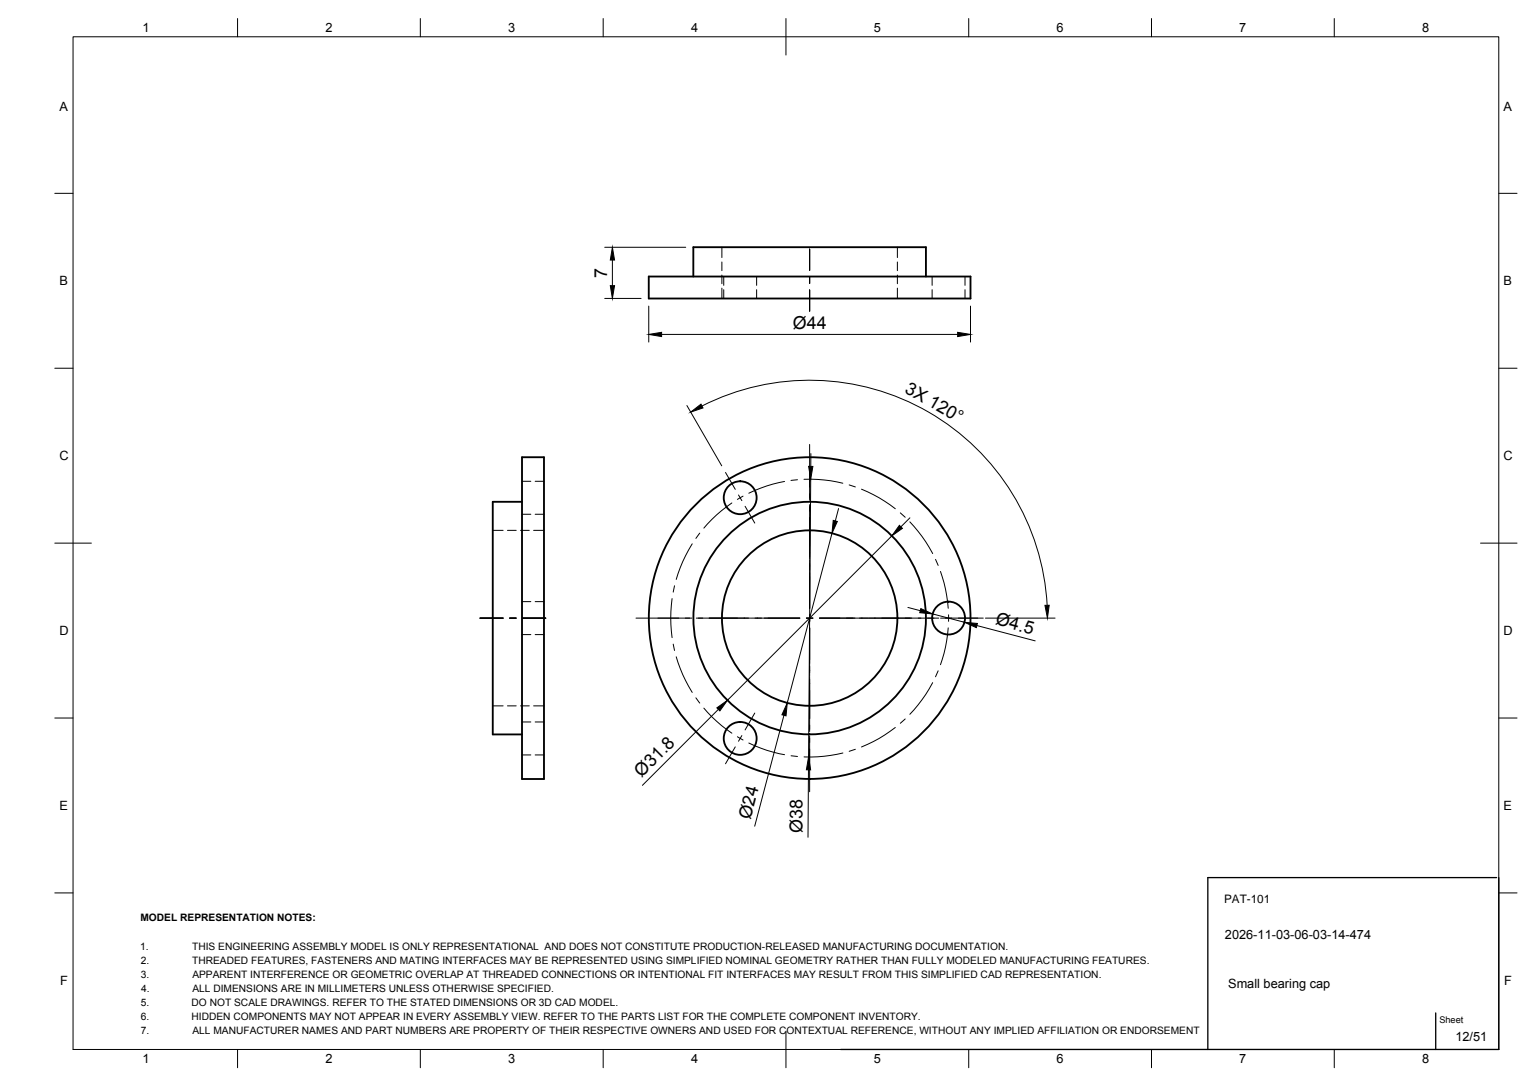
ISO-10303-21;
HEADER;
/* Generated by software containing ST-Developer
 * from STEP Tools, Inc. (www.steptools.com) 
 */

FILE_DESCRIPTION(
/* description */ ('Spur gear reduction stage 2-1 on bearing plates'),
/* implementation_level */ '2;1');

FILE_NAME(
/* name */ 'Small bearing cap.step',
/* time_stamp */ '2026-10-28T03:22:07-07:00',
/* author */ (''),
/* organization */ (''),
/* preprocessor_version */ 'ST-DEVELOPER v20.2',
/* originating_system */ 'Autodesk Translation Framework v15.17.0.0',
/* authorisation */ '');

FILE_SCHEMA (('AUTOMOTIVE_DESIGN { 1 0 10303 214 3 1 1 }'));
ENDSEC;

DATA;
#10=MECHANICAL_DESIGN_GEOMETRIC_PRESENTATION_REPRESENTATION('',(#954),#53909);
#868=SHAPE_REPRESENTATION_RELATIONSHIP('SRR','None',#54095,#911);
#911=ADVANCED_BREP_SHAPE_REPRESENTATION('',(#1012),#53869);
#954=STYLED_ITEM('',(#54397),#1012);
#1012=MANIFOLD_SOLID_BREP('Body1',#11278);
#1140=FACE_BOUND('',#2330,.T.);
#1141=FACE_BOUND('',#2334,.T.);
#1142=FACE_BOUND('',#2335,.T.);
#1143=FACE_BOUND('',#2336,.T.);
#1144=FACE_BOUND('',#2337,.T.);
#1145=FACE_BOUND('',#2339,.T.);
#1146=FACE_BOUND('',#2340,.T.);
#1147=FACE_BOUND('',#2341,.T.);
#1148=FACE_BOUND('',#2342,.T.);
#1280=PLANE('',#12026);
#1281=PLANE('',#12033);
#1282=PLANE('',#12034);
#1597=FACE_OUTER_BOUND('',#2325,.T.);
#1598=FACE_OUTER_BOUND('',#2326,.T.);
#1599=FACE_OUTER_BOUND('',#2327,.T.);
#1600=FACE_OUTER_BOUND('',#2328,.T.);
#1601=FACE_OUTER_BOUND('',#2329,.T.);
#1602=FACE_OUTER_BOUND('',#2331,.T.);
#1603=FACE_OUTER_BOUND('',#2332,.T.);
#1604=FACE_OUTER_BOUND('',#2333,.T.);
#1605=FACE_OUTER_BOUND('',#2338,.T.);
#2325=EDGE_LOOP('',(#7736,#7737,#7738,#7739));
#2326=EDGE_LOOP('',(#7740,#7741,#7742,#7743));
#2327=EDGE_LOOP('',(#7744,#7745,#7746,#7747));
#2328=EDGE_LOOP('',(#7748,#7749,#7750,#7751));
#2329=EDGE_LOOP('',(#7752));
#2330=EDGE_LOOP('',(#7753));
#2331=EDGE_LOOP('',(#7754,#7755,#7756,#7757));
#2332=EDGE_LOOP('',(#7758,#7759,#7760,#7761));
#2333=EDGE_LOOP('',(#7762));
#2334=EDGE_LOOP('',(#7763));
#2335=EDGE_LOOP('',(#7764));
#2336=EDGE_LOOP('',(#7765));
#2337=EDGE_LOOP('',(#7766));
#2338=EDGE_LOOP('',(#7767));
#2339=EDGE_LOOP('',(#7768));
#2340=EDGE_LOOP('',(#7769));
#2341=EDGE_LOOP('',(#7770));
#2342=EDGE_LOOP('',(#7771));
#3065=LINE('',#16403,#3706);
#3066=LINE('',#16409,#3707);
#3067=LINE('',#16415,#3708);
#3068=LINE('',#16421,#3709);
#3069=LINE('',#16428,#3710);
#3070=LINE('',#16434,#3711);
#3706=VECTOR('',#13490,0.225);
#3707=VECTOR('',#13497,0.225);
#3708=VECTOR('',#13504,0.225);
#3709=VECTOR('',#13511,1.59);
#3710=VECTOR('',#13520,1.2);
#3711=VECTOR('',#13527,2.2);
#4363=CIRCLE('',#12015,0.225);
#4364=CIRCLE('',#12016,0.225);
#4365=CIRCLE('',#12018,0.225);
#4366=CIRCLE('',#12019,0.225);
#4367=CIRCLE('',#12021,0.225);
#4368=CIRCLE('',#12022,0.225);
#4369=CIRCLE('',#12024,1.59);
#4370=CIRCLE('',#12025,1.59);
#4371=CIRCLE('',#12027,1.2);
#4372=CIRCLE('',#12029,1.2);
#4373=CIRCLE('',#12031,2.2);
#4374=CIRCLE('',#12032,2.2);
#4912=VERTEX_POINT('',#16400);
#4913=VERTEX_POINT('',#16402);
#4914=VERTEX_POINT('',#16406);
#4915=VERTEX_POINT('',#16408);
#4916=VERTEX_POINT('',#16412);
#4917=VERTEX_POINT('',#16414);
#4918=VERTEX_POINT('',#16418);
#4919=VERTEX_POINT('',#16420);
#4920=VERTEX_POINT('',#16424);
#4921=VERTEX_POINT('',#16427);
#4922=VERTEX_POINT('',#16431);
#4923=VERTEX_POINT('',#16433);
#6010=EDGE_CURVE('',#4912,#4912,#4363,.T.);
#6011=EDGE_CURVE('',#4912,#4913,#3065,.T.);
#6012=EDGE_CURVE('',#4913,#4913,#4364,.T.);
#6013=EDGE_CURVE('',#4914,#4914,#4365,.T.);
#6014=EDGE_CURVE('',#4914,#4915,#3066,.T.);
#6015=EDGE_CURVE('',#4915,#4915,#4366,.T.);
#6016=EDGE_CURVE('',#4916,#4916,#4367,.T.);
#6017=EDGE_CURVE('',#4916,#4917,#3067,.T.);
#6018=EDGE_CURVE('',#4917,#4917,#4368,.T.);
#6019=EDGE_CURVE('',#4918,#4918,#4369,.T.);
#6020=EDGE_CURVE('',#4918,#4919,#3068,.T.);
#6021=EDGE_CURVE('',#4919,#4919,#4370,.T.);
#6022=EDGE_CURVE('',#4920,#4920,#4371,.T.);
#6023=EDGE_CURVE('',#4920,#4921,#3069,.T.);
#6024=EDGE_CURVE('',#4921,#4921,#4372,.T.);
#6025=EDGE_CURVE('',#4922,#4922,#4373,.T.);
#6026=EDGE_CURVE('',#4922,#4923,#3070,.T.);
#6027=EDGE_CURVE('',#4923,#4923,#4374,.T.);
#7736=ORIENTED_EDGE('',*,*,#6010,.F.);
#7737=ORIENTED_EDGE('',*,*,#6011,.T.);
#7738=ORIENTED_EDGE('',*,*,#6012,.F.);
#7739=ORIENTED_EDGE('',*,*,#6011,.F.);
#7740=ORIENTED_EDGE('',*,*,#6013,.F.);
#7741=ORIENTED_EDGE('',*,*,#6014,.T.);
#7742=ORIENTED_EDGE('',*,*,#6015,.F.);
#7743=ORIENTED_EDGE('',*,*,#6014,.F.);
#7744=ORIENTED_EDGE('',*,*,#6016,.F.);
#7745=ORIENTED_EDGE('',*,*,#6017,.T.);
#7746=ORIENTED_EDGE('',*,*,#6018,.F.);
#7747=ORIENTED_EDGE('',*,*,#6017,.F.);
#7748=ORIENTED_EDGE('',*,*,#6019,.F.);
#7749=ORIENTED_EDGE('',*,*,#6020,.T.);
#7750=ORIENTED_EDGE('',*,*,#6021,.F.);
#7751=ORIENTED_EDGE('',*,*,#6020,.F.);
#7752=ORIENTED_EDGE('',*,*,#6019,.T.);
#7753=ORIENTED_EDGE('',*,*,#6022,.T.);
#7754=ORIENTED_EDGE('',*,*,#6022,.F.);
#7755=ORIENTED_EDGE('',*,*,#6023,.T.);
#7756=ORIENTED_EDGE('',*,*,#6024,.T.);
#7757=ORIENTED_EDGE('',*,*,#6023,.F.);
#7758=ORIENTED_EDGE('',*,*,#6025,.F.);
#7759=ORIENTED_EDGE('',*,*,#6026,.T.);
#7760=ORIENTED_EDGE('',*,*,#6027,.T.);
#7761=ORIENTED_EDGE('',*,*,#6026,.F.);
#7762=ORIENTED_EDGE('',*,*,#6025,.T.);
#7763=ORIENTED_EDGE('',*,*,#6012,.T.);
#7764=ORIENTED_EDGE('',*,*,#6015,.T.);
#7765=ORIENTED_EDGE('',*,*,#6018,.T.);
#7766=ORIENTED_EDGE('',*,*,#6021,.T.);
#7767=ORIENTED_EDGE('',*,*,#6027,.F.);
#7768=ORIENTED_EDGE('',*,*,#6010,.T.);
#7769=ORIENTED_EDGE('',*,*,#6013,.T.);
#7770=ORIENTED_EDGE('',*,*,#6016,.T.);
#7771=ORIENTED_EDGE('',*,*,#6024,.F.);
#10472=CYLINDRICAL_SURFACE('',#12014,0.225);
#10473=CYLINDRICAL_SURFACE('',#12017,0.225);
#10474=CYLINDRICAL_SURFACE('',#12020,0.225);
#10475=CYLINDRICAL_SURFACE('',#12023,1.59);
#10476=CYLINDRICAL_SURFACE('',#12028,1.2);
#10477=CYLINDRICAL_SURFACE('',#12030,2.2);
#10717=ADVANCED_FACE('',(#1597),#10472,.F.);
#10718=ADVANCED_FACE('',(#1598),#10473,.F.);
#10719=ADVANCED_FACE('',(#1599),#10474,.F.);
#10720=ADVANCED_FACE('',(#1600),#10475,.T.);
#10721=ADVANCED_FACE('',(#1601,#1140),#1280,.T.);
#10722=ADVANCED_FACE('',(#1602),#10476,.F.);
#10723=ADVANCED_FACE('',(#1603),#10477,.T.);
#10724=ADVANCED_FACE('',(#1604,#1141,#1142,#1143,#1144),#1281,.T.);
#10725=ADVANCED_FACE('',(#1605,#1145,#1146,#1147,#1148),#1282,.F.);
#11278=CLOSED_SHELL('',(#10717,#10718,#10719,#10720,#10721,#10722,#10723,
#10724,#10725));
#12013=AXIS2_PLACEMENT_3D('',#16398,#13484,#13485);
#12014=AXIS2_PLACEMENT_3D('',#16399,#13486,#13487);
#12015=AXIS2_PLACEMENT_3D('',#16401,#13488,#13489);
#12016=AXIS2_PLACEMENT_3D('',#16404,#13491,#13492);
#12017=AXIS2_PLACEMENT_3D('',#16405,#13493,#13494);
#12018=AXIS2_PLACEMENT_3D('',#16407,#13495,#13496);
#12019=AXIS2_PLACEMENT_3D('',#16410,#13498,#13499);
#12020=AXIS2_PLACEMENT_3D('',#16411,#13500,#13501);
#12021=AXIS2_PLACEMENT_3D('',#16413,#13502,#13503);
#12022=AXIS2_PLACEMENT_3D('',#16416,#13505,#13506);
#12023=AXIS2_PLACEMENT_3D('',#16417,#13507,#13508);
#12024=AXIS2_PLACEMENT_3D('',#16419,#13509,#13510);
#12025=AXIS2_PLACEMENT_3D('',#16422,#13512,#13513);
#12026=AXIS2_PLACEMENT_3D('',#16423,#13514,#13515);
#12027=AXIS2_PLACEMENT_3D('',#16425,#13516,#13517);
#12028=AXIS2_PLACEMENT_3D('',#16426,#13518,#13519);
#12029=AXIS2_PLACEMENT_3D('',#16429,#13521,#13522);
#12030=AXIS2_PLACEMENT_3D('',#16430,#13523,#13524);
#12031=AXIS2_PLACEMENT_3D('',#16432,#13525,#13526);
#12032=AXIS2_PLACEMENT_3D('',#16435,#13528,#13529);
#12033=AXIS2_PLACEMENT_3D('',#16436,#13530,#13531);
#12034=AXIS2_PLACEMENT_3D('',#16437,#13532,#13533);
#13484=DIRECTION('axis',(0.,0.,1.));
#13485=DIRECTION('refdir',(1.,0.,0.));
#13486=DIRECTION('center_axis',(0.,1.,0.));
#13487=DIRECTION('ref_axis',(1.,0.,0.));
#13488=DIRECTION('center_axis',(0.,1.,0.));
#13489=DIRECTION('ref_axis',(1.,0.,0.));
#13490=DIRECTION('',(0.,1.,0.));
#13491=DIRECTION('center_axis',(0.,-1.,0.));
#13492=DIRECTION('ref_axis',(1.,0.,0.));
#13493=DIRECTION('center_axis',(0.,1.,0.));
#13494=DIRECTION('ref_axis',(1.,0.,0.));
#13495=DIRECTION('center_axis',(0.,1.,0.));
#13496=DIRECTION('ref_axis',(1.,0.,0.));
#13497=DIRECTION('',(0.,1.,0.));
#13498=DIRECTION('center_axis',(0.,-1.,0.));
#13499=DIRECTION('ref_axis',(1.,0.,0.));
#13500=DIRECTION('center_axis',(0.,1.,0.));
#13501=DIRECTION('ref_axis',(1.,0.,0.));
#13502=DIRECTION('center_axis',(0.,1.,0.));
#13503=DIRECTION('ref_axis',(1.,0.,0.));
#13504=DIRECTION('',(0.,1.,0.));
#13505=DIRECTION('center_axis',(0.,-1.,0.));
#13506=DIRECTION('ref_axis',(1.,0.,0.));
#13507=DIRECTION('center_axis',(0.,1.,0.));
#13508=DIRECTION('ref_axis',(1.,0.,0.));
#13509=DIRECTION('center_axis',(0.,1.,0.));
#13510=DIRECTION('ref_axis',(1.,0.,0.));
#13511=DIRECTION('',(0.,-1.,0.));
#13512=DIRECTION('center_axis',(0.,-1.,0.));
#13513=DIRECTION('ref_axis',(1.,0.,0.));
#13514=DIRECTION('center_axis',(0.,1.,0.));
#13515=DIRECTION('ref_axis',(1.,0.,0.));
#13516=DIRECTION('center_axis',(0.,-1.,0.));
#13517=DIRECTION('ref_axis',(1.,0.,0.));
#13518=DIRECTION('center_axis',(0.,1.,0.));
#13519=DIRECTION('ref_axis',(1.,0.,0.));
#13520=DIRECTION('',(0.,-1.,0.));
#13521=DIRECTION('center_axis',(0.,-1.,0.));
#13522=DIRECTION('ref_axis',(1.,0.,0.));
#13523=DIRECTION('center_axis',(0.,1.,0.));
#13524=DIRECTION('ref_axis',(1.,0.,0.));
#13525=DIRECTION('center_axis',(0.,1.,0.));
#13526=DIRECTION('ref_axis',(1.,0.,0.));
#13527=DIRECTION('',(0.,-1.,0.));
#13528=DIRECTION('center_axis',(0.,1.,0.));
#13529=DIRECTION('ref_axis',(1.,0.,0.));
#13530=DIRECTION('center_axis',(0.,1.,0.));
#13531=DIRECTION('ref_axis',(1.,0.,0.));
#13532=DIRECTION('center_axis',(0.,1.,0.));
#13533=DIRECTION('ref_axis',(1.,0.,0.));
#16398=CARTESIAN_POINT('',(0.,0.,0.));
#16399=CARTESIAN_POINT('Origin',(1.16341445918999E-16,-4.8,6.9));
#16400=CARTESIAN_POINT('',(-0.225,-4.7,6.9));
#16401=CARTESIAN_POINT('Origin',(1.16341445918999E-16,-4.7,6.9));
#16402=CARTESIAN_POINT('',(-0.225,-4.4,6.9));
#16403=CARTESIAN_POINT('',(-0.225,-4.8,6.9));
#16404=CARTESIAN_POINT('Origin',(1.16341445918999E-16,-4.4,6.9));
#16405=CARTESIAN_POINT('Origin',(-1.64544826719043,-4.8,4.05));
#16406=CARTESIAN_POINT('',(-1.87044826719043,-4.7,4.05));
#16407=CARTESIAN_POINT('Origin',(-1.64544826719043,-4.7,4.05));
#16408=CARTESIAN_POINT('',(-1.87044826719043,-4.4,4.05));
#16409=CARTESIAN_POINT('',(-1.87044826719043,-4.8,4.05));
#16410=CARTESIAN_POINT('Origin',(-1.64544826719043,-4.4,4.05));
#16411=CARTESIAN_POINT('Origin',(1.64544826719043,-4.8,4.05));
#16412=CARTESIAN_POINT('',(1.42044826719043,-4.7,4.05));
#16413=CARTESIAN_POINT('Origin',(1.64544826719043,-4.7,4.05));
#16414=CARTESIAN_POINT('',(1.42044826719043,-4.4,4.05));
#16415=CARTESIAN_POINT('',(1.42044826719043,-4.8,4.05));
#16416=CARTESIAN_POINT('Origin',(1.64544826719043,-4.4,4.05));
#16417=CARTESIAN_POINT('Origin',(0.,-4.4,5.));
#16418=CARTESIAN_POINT('',(-1.59,-4.,5.));
#16419=CARTESIAN_POINT('Origin',(0.,-4.,5.));
#16420=CARTESIAN_POINT('',(-1.59,-4.4,5.));
#16421=CARTESIAN_POINT('',(-1.59,-4.4,5.));
#16422=CARTESIAN_POINT('Origin',(0.,-4.4,5.));
#16423=CARTESIAN_POINT('Origin',(0.,-4.,5.));
#16424=CARTESIAN_POINT('',(-1.2,-4.,5.));
#16425=CARTESIAN_POINT('Origin',(0.,-4.,5.));
#16426=CARTESIAN_POINT('Origin',(0.,-4.7,5.));
#16427=CARTESIAN_POINT('',(-1.2,-4.7,5.));
#16428=CARTESIAN_POINT('',(-1.2,-4.7,5.));
#16429=CARTESIAN_POINT('Origin',(0.,-4.7,5.));
#16430=CARTESIAN_POINT('Origin',(0.,-4.7,5.));
#16431=CARTESIAN_POINT('',(-2.2,-4.4,5.));
#16432=CARTESIAN_POINT('Origin',(0.,-4.4,5.));
#16433=CARTESIAN_POINT('',(-2.2,-4.7,5.));
#16434=CARTESIAN_POINT('',(-2.2,-4.7,5.));
#16435=CARTESIAN_POINT('Origin',(0.,-4.7,5.));
#16436=CARTESIAN_POINT('Origin',(0.,-4.4,5.));
#16437=CARTESIAN_POINT('Origin',(0.,-4.7,5.));
#53819=UNCERTAINTY_MEASURE_WITH_UNIT(LENGTH_MEASURE(0.001),#53910,
'DISTANCE_ACCURACY_VALUE',
'Maximum model space distance between geometric entities at asserted c
onnectivities');
#53859=UNCERTAINTY_MEASURE_WITH_UNIT(LENGTH_MEASURE(0.001),#53910,
'DISTANCE_ACCURACY_VALUE',
'Maximum model space distance between geometric entities at asserted c
onnectivities');
#53869=(
GEOMETRIC_REPRESENTATION_CONTEXT(3)
GLOBAL_UNCERTAINTY_ASSIGNED_CONTEXT((#53819))
GLOBAL_UNIT_ASSIGNED_CONTEXT((#53910,#53912,#53913))
REPRESENTATION_CONTEXT('','3D')
);
#53909=(
GEOMETRIC_REPRESENTATION_CONTEXT(3)
GLOBAL_UNCERTAINTY_ASSIGNED_CONTEXT((#53859))
GLOBAL_UNIT_ASSIGNED_CONTEXT((#53910,#53912,#53913))
REPRESENTATION_CONTEXT('','3D')
);
#53910=(
LENGTH_UNIT()
NAMED_UNIT(*)
SI_UNIT(.CENTI.,.METRE.)
);
#53912=(
NAMED_UNIT(*)
PLANE_ANGLE_UNIT()
SI_UNIT($,.RADIAN.)
);
#53913=(
NAMED_UNIT(*)
SI_UNIT($,.STERADIAN.)
SOLID_ANGLE_UNIT()
);
#53923=SHAPE_DEFINITION_REPRESENTATION(#53972,#54095);
#53972=PRODUCT_DEFINITION_SHAPE('',$,#54145);
#54095=SHAPE_REPRESENTATION('',(#12013),#53869);
#54135=PRODUCT_DEFINITION_CONTEXT('part definition',#54284,'design');
#54145=PRODUCT_DEFINITION('Small bearing cap','Small bearing cap',#54194,
#54135);
#54194=PRODUCT_DEFINITION_FORMATION('',$,#54295);
#54284=APPLICATION_CONTEXT(
'Core Data for Automotive Mechanical Design Process');
#54285=PRODUCT_CONTEXT('part definition',#54284,'mechanical');
#54295=PRODUCT('Small bearing cap','Small bearing cap',
'Small bearing cap',(#54285));
#54391=COLOUR_RGB('Grey',0.48,0.52,0.57);
#54392=FILL_AREA_STYLE_COLOUR('',#54391);
#54393=FILL_AREA_STYLE('',(#54392));
#54394=SURFACE_STYLE_FILL_AREA(#54393);
#54395=SURFACE_SIDE_STYLE('',(#54394));
#54396=SURFACE_STYLE_USAGE(.BOTH.,#54395);
#54397=PRESENTATION_STYLE_ASSIGNMENT((#54396));
ENDSEC;
END-ISO-10303-21;
